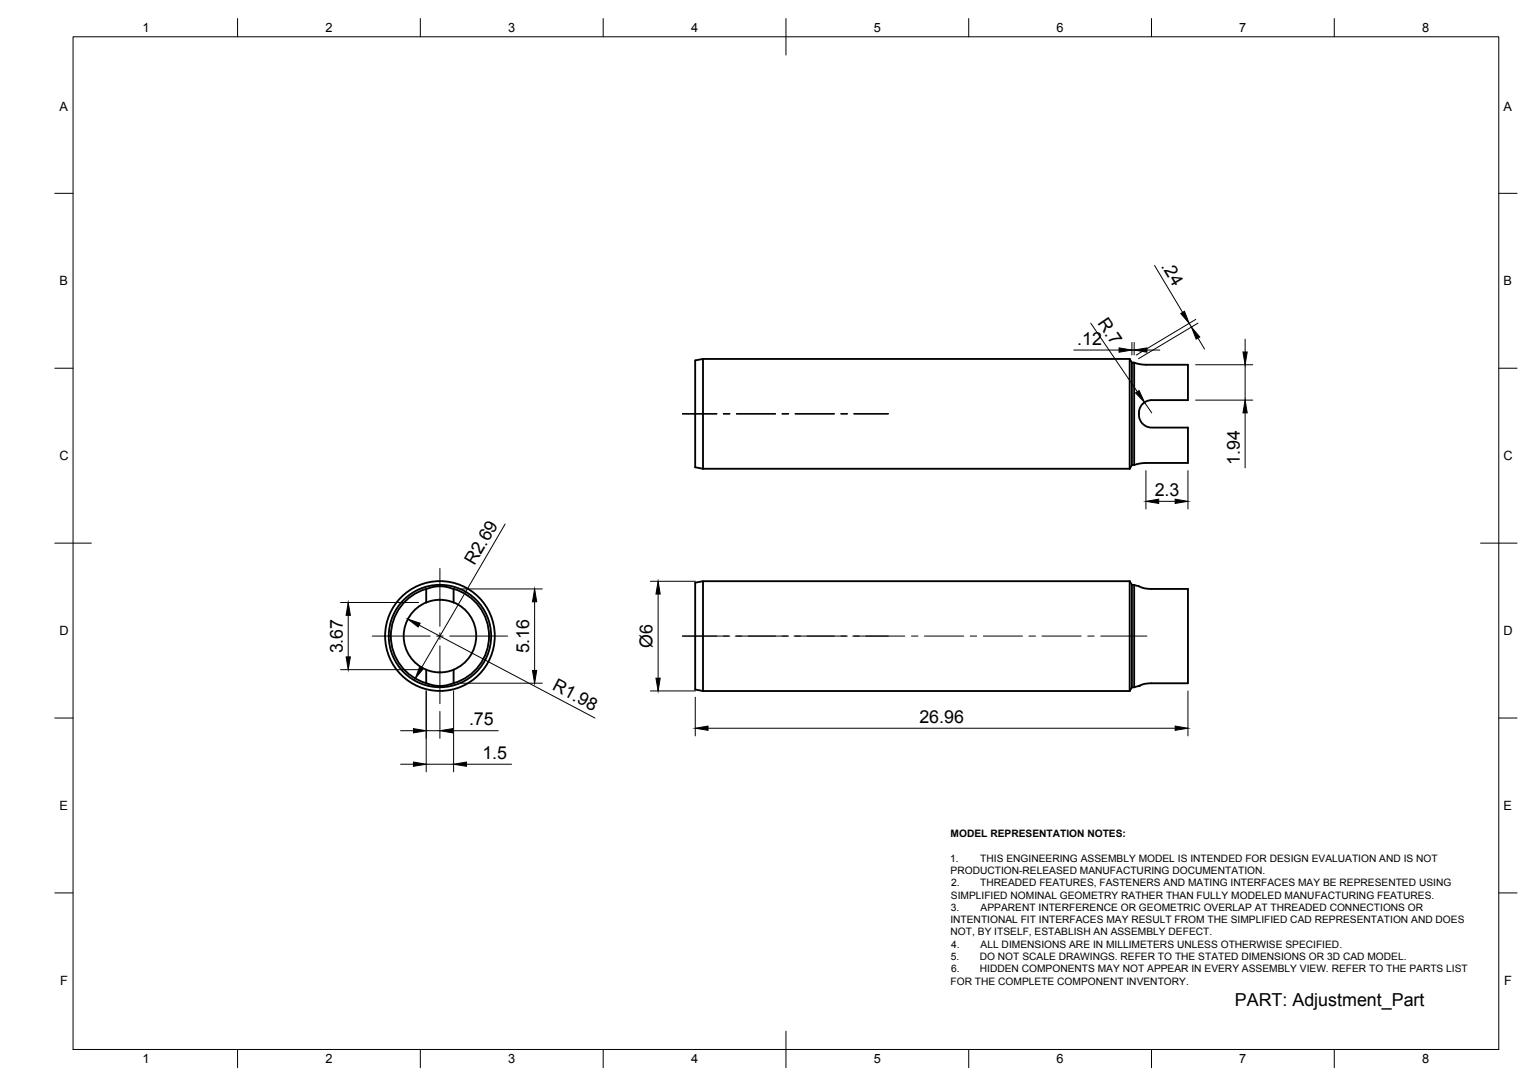
ISO-10303-21;
HEADER;
/* Generated by software containing ST-Developer
 * from STEP Tools, Inc. (www.steptools.com) 
 */

FILE_DESCRIPTION(
/* description */ (''),
/* implementation_level */ '2;1');

FILE_NAME(
/* name */ 'Adjustment_Part.step',
/* time_stamp */ '2026-10-05T00:51:14-07:00',
/* author */ (''),
/* organization */ (''),
/* preprocessor_version */ 'ST-DEVELOPER v20.2',
/* originating_system */ 'Autodesk Translation Framework v15.15.0.0',
/* authorisation */ '');

FILE_SCHEMA (('AUTOMOTIVE_DESIGN { 1 0 10303 214 3 1 1 }'));
ENDSEC;

DATA;
#10=MECHANICAL_DESIGN_GEOMETRIC_PRESENTATION_REPRESENTATION('',(#393),#4613);
#43=TOROIDAL_SURFACE('',#1858,4.57788729236058,1.89228053659161);
#64=CONICAL_SURFACE('',#1877,2.89950556638236,1.03144708645266);
#65=CONICAL_SURFACE('',#1881,2.96124530227324,0.181516066311168);
#89=FACE_BOUND('',#627,.T.);
#90=FACE_BOUND('',#633,.T.);
#120=PLANE('',#1842);
#121=PLANE('',#1843);
#122=PLANE('',#1845);
#123=PLANE('',#1848);
#124=PLANE('',#1850);
#125=PLANE('',#1852);
#126=PLANE('',#1871);
#127=PLANE('',#1872);
#128=PLANE('',#1873);
#129=PLANE('',#1883);
#153=B_SPLINE_CURVE_WITH_KNOTS('',3,(#4375,#4376,#4377,#4378,#4379,#4380),
 .UNSPECIFIED.,.F.,.F.,(4,2,4),(0.,0.0265093466366244,0.0315326488828016),
 .UNSPECIFIED.);
#154=B_SPLINE_CURVE_WITH_KNOTS('',3,(#4382,#4383,#4384,#4385,#4386,#4387,
#4388,#4389,#4390,#4391),.UNSPECIFIED.,.F.,.F.,(4,2,2,2,4),(-0.106715130399001,
-0.0799992414062105,-0.0532833524134197,-0.0266416762067098,0.),
 .UNSPECIFIED.);
#155=B_SPLINE_CURVE_WITH_KNOTS('',3,(#4394,#4395,#4396,#4397,#4398,#4399,
#4400,#4401,#4402,#4403,#4404,#4405,#4406),.UNSPECIFIED.,.F.,.F.,(4,2,2,
2,3,4),(0.378639974335924,0.39855724329992,0.425776827887283,0.447703205216881,
0.457107149533339,0.457130414187804),.UNSPECIFIED.);
#156=B_SPLINE_CURVE_WITH_KNOTS('',3,(#4424,#4425,#4426,#4427,#4428,#4429,
#4430,#4431,#4432,#4433,#4434,#4435,#4436),.UNSPECIFIED.,.F.,.F.,(4,3,2,
2,2,4),(0.457052713610798,0.457075978112808,0.477097828431014,0.502267294711213,
0.530728459336765,0.53557163395288),.UNSPECIFIED.);
#157=B_SPLINE_CURVE_WITH_KNOTS('',3,(#4437,#4438,#4439,#4440,#4441,#4442,
#4443,#4444,#4445,#4446),.UNSPECIFIED.,.F.,.F.,(4,2,2,2,4),(-0.212983885016079,
-0.186342208809369,-0.159700532602659,-0.132984643609868,-0.106268754617077),
 .UNSPECIFIED.);
#158=B_SPLINE_CURVE_WITH_KNOTS('',3,(#4447,#4448,#4449,#4450,#4451,#4452),
 .UNSPECIFIED.,.F.,.F.,(4,2,4),(0.180491212128822,0.185514514374999,0.212023861011624),
 .UNSPECIFIED.);
#159=B_SPLINE_CURVE_WITH_KNOTS('',3,(#4465,#4466,#4467,#4468,#4469,#4470,
#4471,#4472,#4473,#4474),.UNSPECIFIED.,.F.,.F.,(4,2,2,2,4),(0.152701408415346,
0.169165149472481,0.195857989456366,0.218518872787138,0.230918738867668),
 .UNSPECIFIED.);
#160=B_SPLINE_CURVE_WITH_KNOTS('',3,(#4475,#4476,#4477,#4478,#4479,#4480),
 .UNSPECIFIED.,.F.,.F.,(4,2,4),(0.212023861011624,0.238533207648248,0.243556509894426),
 .UNSPECIFIED.);
#161=B_SPLINE_CURVE_WITH_KNOTS('',3,(#4482,#4483,#4484,#4485,#4486,#4487,
#4488,#4489,#4490,#4491),.UNSPECIFIED.,.F.,.F.,(4,2,2,2,4),(-0.319699015415081,
-0.29298312642229,-0.266267237429499,-0.239625561222789,-0.212983885016079),
 .UNSPECIFIED.);
#162=B_SPLINE_CURVE_WITH_KNOTS('',3,(#4505,#4506,#4507,#4508,#4509,#4510),
 .UNSPECIFIED.,.F.,.F.,(4,2,4),(0.392515073140443,0.39753837538662,0.424047722023245),
 .UNSPECIFIED.);
#163=B_SPLINE_CURVE_WITH_KNOTS('',3,(#4511,#4512,#4513,#4514,#4515,#4516,
#4517,#4518,#4519,#4520),.UNSPECIFIED.,.F.,.F.,(4,2,2,2,4),(0.224352648954622,
0.240815002701601,0.264724046908964,0.293460711591788,0.30255788453281),
 .UNSPECIFIED.);
#164=B_SPLINE_CURVE_WITH_KNOTS('',3,(#4521,#4522,#4523,#4524,#4525,#4526,
#4527,#4528,#4529,#4530),.UNSPECIFIED.,.F.,.F.,(4,2,2,2,4),(-0.425967770032155,
-0.399326093825445,-0.372684417618735,-0.345968528625944,-0.319252639633153),
 .UNSPECIFIED.);
#220=LINE('',#4358,#303);
#221=LINE('',#4360,#304);
#222=LINE('',#4362,#305);
#223=LINE('',#4363,#306);
#224=LINE('',#4367,#307);
#225=LINE('',#4369,#308);
#226=LINE('',#4371,#309);
#227=LINE('',#4372,#310);
#228=LINE('',#4393,#311);
#229=LINE('',#4412,#312);
#230=LINE('',#4416,#313);
#231=LINE('',#4418,#314);
#232=LINE('',#4420,#315);
#233=LINE('',#4421,#316);
#234=LINE('',#4456,#317);
#235=LINE('',#4458,#318);
#236=LINE('',#4460,#319);
#237=LINE('',#4461,#320);
#238=LINE('',#4492,#321);
#239=LINE('',#4501,#322);
#240=LINE('',#4539,#323);
#241=LINE('',#4555,#324);
#242=LINE('',#4559,#325);
#243=LINE('',#4563,#326);
#244=LINE('',#4566,#327);
#245=LINE('',#4572,#328);
#303=VECTOR('',#2261,10.);
#304=VECTOR('',#2262,10.);
#305=VECTOR('',#2263,10.);
#306=VECTOR('',#2264,10.);
#307=VECTOR('',#2267,10.);
#308=VECTOR('',#2268,10.);
#309=VECTOR('',#2269,10.);
#310=VECTOR('',#2270,10.);
#311=VECTOR('',#2273,10.);
#312=VECTOR('',#2280,10.);
#313=VECTOR('',#2283,10.);
#314=VECTOR('',#2284,10.);
#315=VECTOR('',#2285,10.);
#316=VECTOR('',#2286,10.);
#317=VECTOR('',#2291,10.);
#318=VECTOR('',#2292,10.);
#319=VECTOR('',#2293,10.);
#320=VECTOR('',#2294,10.);
#321=VECTOR('',#2297,10.);
#322=VECTOR('',#2306,10.);
#323=VECTOR('',#2323,1.9840612380693);
#324=VECTOR('',#2350,2.79839874569029);
#325=VECTOR('',#2355,2.89950556638236);
#326=VECTOR('',#2360,3.00061238707443);
#327=VECTOR('',#2363,2.96124530227324);
#328=VECTOR('',#2372,2.3164003912567);
#360=CYLINDRICAL_SURFACE('',#1844,0.699999999999994);
#361=CYLINDRICAL_SURFACE('',#1849,0.699999999999998);
#362=CYLINDRICAL_SURFACE('',#1851,0.699999999999998);
#363=CYLINDRICAL_SURFACE('',#1857,0.699999999999994);
#364=CYLINDRICAL_SURFACE('',#1863,1.9840612380693);
#365=CYLINDRICAL_SURFACE('',#1867,2.68560675576897);
#366=CYLINDRICAL_SURFACE('',#1869,2.68560675576897);
#367=CYLINDRICAL_SURFACE('',#1875,2.79839874569029);
#368=CYLINDRICAL_SURFACE('',#1879,3.00061238707443);
#369=CYLINDRICAL_SURFACE('',#1885,2.3164003912567);
#377=SHAPE_REPRESENTATION_RELATIONSHIP('SRR','None',#4651,#385);
#385=ADVANCED_BREP_SHAPE_REPRESENTATION('',(#401),#4611);
#393=STYLED_ITEM('',(#4695),#401);
#401=MANIFOLD_SOLID_BREP('Body1',#1600);
#482=FACE_OUTER_BOUND('',#610,.T.);
#483=FACE_OUTER_BOUND('',#611,.T.);
#484=FACE_OUTER_BOUND('',#612,.T.);
#485=FACE_OUTER_BOUND('',#613,.T.);
#486=FACE_OUTER_BOUND('',#614,.T.);
#487=FACE_OUTER_BOUND('',#615,.T.);
#488=FACE_OUTER_BOUND('',#616,.T.);
#489=FACE_OUTER_BOUND('',#617,.T.);
#490=FACE_OUTER_BOUND('',#618,.T.);
#491=FACE_OUTER_BOUND('',#619,.T.);
#492=FACE_OUTER_BOUND('',#620,.T.);
#493=FACE_OUTER_BOUND('',#621,.T.);
#494=FACE_OUTER_BOUND('',#622,.T.);
#495=FACE_OUTER_BOUND('',#623,.T.);
#496=FACE_OUTER_BOUND('',#624,.T.);
#497=FACE_OUTER_BOUND('',#625,.T.);
#498=FACE_OUTER_BOUND('',#626,.T.);
#499=FACE_OUTER_BOUND('',#628,.T.);
#500=FACE_OUTER_BOUND('',#629,.T.);
#501=FACE_OUTER_BOUND('',#630,.T.);
#502=FACE_OUTER_BOUND('',#631,.T.);
#503=FACE_OUTER_BOUND('',#632,.T.);
#504=FACE_OUTER_BOUND('',#634,.T.);
#610=EDGE_LOOP('',(#1359,#1360,#1361,#1362));
#611=EDGE_LOOP('',(#1363,#1364,#1365,#1366));
#612=EDGE_LOOP('',(#1367,#1368,#1369,#1370,#1371));
#613=EDGE_LOOP('',(#1372,#1373,#1374,#1375));
#614=EDGE_LOOP('',(#1376,#1377,#1378,#1379));
#615=EDGE_LOOP('',(#1380,#1381,#1382,#1383,#1384));
#616=EDGE_LOOP('',(#1385,#1386,#1387,#1388));
#617=EDGE_LOOP('',(#1389,#1390,#1391,#1392,#1393));
#618=EDGE_LOOP('',(#1394,#1395,#1396,#1397,#1398,#1399));
#619=EDGE_LOOP('',(#1400,#1401,#1402,#1403,#1404));
#620=EDGE_LOOP('',(#1405,#1406,#1407,#1408,#1409,#1410,#1411,#1412,#1413,
#1414,#1415,#1416));
#621=EDGE_LOOP('',(#1417,#1418,#1419,#1420,#1421,#1422,#1423,#1424,#1425,
#1426,#1427,#1428,#1429,#1430,#1431,#1432));
#622=EDGE_LOOP('',(#1433,#1434,#1435,#1436,#1437,#1438));
#623=EDGE_LOOP('',(#1439,#1440,#1441,#1442,#1443,#1444));
#624=EDGE_LOOP('',(#1445,#1446,#1447,#1448));
#625=EDGE_LOOP('',(#1449,#1450,#1451,#1452));
#626=EDGE_LOOP('',(#1453));
#627=EDGE_LOOP('',(#1454));
#628=EDGE_LOOP('',(#1455,#1456,#1457,#1458));
#629=EDGE_LOOP('',(#1459,#1460,#1461,#1462));
#630=EDGE_LOOP('',(#1463,#1464,#1465,#1466));
#631=EDGE_LOOP('',(#1467,#1468,#1469,#1470));
#632=EDGE_LOOP('',(#1471));
#633=EDGE_LOOP('',(#1472));
#634=EDGE_LOOP('',(#1473,#1474,#1475,#1476));
#707=CIRCLE('',#1846,2.7248783394621);
#708=CIRCLE('',#1847,1.9840612380693);
#709=CIRCLE('',#1853,2.7248783394621);
#710=CIRCLE('',#1854,1.9840612380693);
#711=CIRCLE('',#1855,1.9840612380693);
#712=CIRCLE('',#1856,2.7248783394621);
#713=CIRCLE('',#1859,2.79839874569029);
#714=CIRCLE('',#1860,1.89228053659161);
#715=CIRCLE('',#1861,2.68560675576897);
#716=CIRCLE('',#1862,2.68560675576897);
#717=CIRCLE('',#1864,1.9840612380693);
#718=CIRCLE('',#1865,1.9840612380693);
#719=CIRCLE('',#1866,1.9840612380693);
#720=CIRCLE('',#1868,2.68560675576897);
#721=CIRCLE('',#1870,2.68560675576897);
#722=CIRCLE('',#1874,2.3164003912567);
#723=CIRCLE('',#1876,2.79839874569029);
#724=CIRCLE('',#1878,3.00061238707443);
#725=CIRCLE('',#1880,3.00061238707443);
#726=CIRCLE('',#1882,2.92187821747206);
#727=CIRCLE('',#1884,2.3164003912567);
#822=VERTEX_POINT('',#4356);
#823=VERTEX_POINT('',#4357);
#824=VERTEX_POINT('',#4359);
#825=VERTEX_POINT('',#4361);
#826=VERTEX_POINT('',#4365);
#827=VERTEX_POINT('',#4366);
#828=VERTEX_POINT('',#4368);
#829=VERTEX_POINT('',#4370);
#830=VERTEX_POINT('',#4374);
#831=VERTEX_POINT('',#4381);
#832=VERTEX_POINT('',#4392);
#833=VERTEX_POINT('',#4408);
#834=VERTEX_POINT('',#4410);
#835=VERTEX_POINT('',#4414);
#836=VERTEX_POINT('',#4415);
#837=VERTEX_POINT('',#4417);
#838=VERTEX_POINT('',#4419);
#839=VERTEX_POINT('',#4423);
#840=VERTEX_POINT('',#4454);
#841=VERTEX_POINT('',#4455);
#842=VERTEX_POINT('',#4457);
#843=VERTEX_POINT('',#4459);
#844=VERTEX_POINT('',#4463);
#845=VERTEX_POINT('',#4464);
#846=VERTEX_POINT('',#4481);
#847=VERTEX_POINT('',#4494);
#848=VERTEX_POINT('',#4496);
#849=VERTEX_POINT('',#4498);
#850=VERTEX_POINT('',#4500);
#851=VERTEX_POINT('',#4504);
#852=VERTEX_POINT('',#4532);
#853=VERTEX_POINT('',#4538);
#854=VERTEX_POINT('',#4550);
#855=VERTEX_POINT('',#4553);
#856=VERTEX_POINT('',#4557);
#857=VERTEX_POINT('',#4561);
#858=VERTEX_POINT('',#4565);
#859=VERTEX_POINT('',#4569);
#1007=EDGE_CURVE('',#822,#823,#220,.T.);
#1008=EDGE_CURVE('',#824,#822,#221,.T.);
#1009=EDGE_CURVE('',#825,#824,#222,.T.);
#1010=EDGE_CURVE('',#825,#823,#223,.T.);
#1011=EDGE_CURVE('',#826,#827,#224,.T.);
#1012=EDGE_CURVE('',#826,#828,#225,.T.);
#1013=EDGE_CURVE('',#829,#828,#226,.T.);
#1014=EDGE_CURVE('',#827,#829,#227,.T.);
#1015=EDGE_CURVE('',#823,#830,#153,.T.);
#1016=EDGE_CURVE('',#831,#825,#154,.T.);
#1017=EDGE_CURVE('',#832,#831,#228,.T.);
#1018=EDGE_CURVE('',#830,#832,#155,.T.);
#1019=EDGE_CURVE('',#832,#833,#707,.T.);
#1020=EDGE_CURVE('',#834,#831,#708,.T.);
#1021=EDGE_CURVE('',#833,#834,#229,.T.);
#1022=EDGE_CURVE('',#835,#836,#230,.T.);
#1023=EDGE_CURVE('',#835,#837,#231,.T.);
#1024=EDGE_CURVE('',#838,#837,#232,.T.);
#1025=EDGE_CURVE('',#836,#838,#233,.T.);
#1026=EDGE_CURVE('',#833,#839,#156,.T.);
#1027=EDGE_CURVE('',#837,#834,#157,.T.);
#1028=EDGE_CURVE('',#839,#835,#158,.T.);
#1029=EDGE_CURVE('',#840,#841,#234,.T.);
#1030=EDGE_CURVE('',#842,#840,#235,.T.);
#1031=EDGE_CURVE('',#843,#842,#236,.T.);
#1032=EDGE_CURVE('',#843,#841,#237,.T.);
#1033=EDGE_CURVE('',#844,#845,#159,.T.);
#1034=EDGE_CURVE('',#841,#844,#160,.T.);
#1035=EDGE_CURVE('',#846,#843,#161,.T.);
#1036=EDGE_CURVE('',#846,#845,#238,.T.);
#1037=EDGE_CURVE('',#845,#847,#709,.T.);
#1038=EDGE_CURVE('',#848,#846,#710,.T.);
#1039=EDGE_CURVE('',#849,#848,#711,.T.);
#1040=EDGE_CURVE('',#849,#850,#239,.T.);
#1041=EDGE_CURVE('',#847,#850,#712,.T.);
#1042=EDGE_CURVE('',#851,#826,#162,.T.);
#1043=EDGE_CURVE('',#850,#851,#163,.T.);
#1044=EDGE_CURVE('',#828,#849,#164,.T.);
#1045=EDGE_CURVE('',#852,#852,#713,.T.);
#1046=EDGE_CURVE('',#852,#847,#714,.T.);
#1047=EDGE_CURVE('',#851,#830,#715,.T.);
#1048=EDGE_CURVE('',#839,#844,#716,.T.);
#1049=EDGE_CURVE('',#848,#853,#240,.T.);
#1050=EDGE_CURVE('',#853,#853,#717,.T.);
#1051=EDGE_CURVE('',#838,#842,#718,.T.);
#1052=EDGE_CURVE('',#829,#824,#719,.T.);
#1053=EDGE_CURVE('',#836,#840,#720,.T.);
#1054=EDGE_CURVE('',#827,#822,#721,.T.);
#1055=EDGE_CURVE('',#854,#854,#722,.T.);
#1056=EDGE_CURVE('',#855,#855,#723,.T.);
#1057=EDGE_CURVE('',#855,#852,#241,.T.);
#1058=EDGE_CURVE('',#856,#856,#724,.T.);
#1059=EDGE_CURVE('',#856,#855,#242,.T.);
#1060=EDGE_CURVE('',#857,#857,#725,.T.);
#1061=EDGE_CURVE('',#857,#856,#243,.T.);
#1062=EDGE_CURVE('',#857,#858,#244,.T.);
#1063=EDGE_CURVE('',#858,#858,#726,.T.);
#1064=EDGE_CURVE('',#859,#859,#727,.T.);
#1065=EDGE_CURVE('',#854,#859,#245,.T.);
#1359=ORIENTED_EDGE('',*,*,#1007,.F.);
#1360=ORIENTED_EDGE('',*,*,#1008,.F.);
#1361=ORIENTED_EDGE('',*,*,#1009,.F.);
#1362=ORIENTED_EDGE('',*,*,#1010,.T.);
#1363=ORIENTED_EDGE('',*,*,#1011,.F.);
#1364=ORIENTED_EDGE('',*,*,#1012,.T.);
#1365=ORIENTED_EDGE('',*,*,#1013,.F.);
#1366=ORIENTED_EDGE('',*,*,#1014,.F.);
#1367=ORIENTED_EDGE('',*,*,#1015,.F.);
#1368=ORIENTED_EDGE('',*,*,#1010,.F.);
#1369=ORIENTED_EDGE('',*,*,#1016,.F.);
#1370=ORIENTED_EDGE('',*,*,#1017,.F.);
#1371=ORIENTED_EDGE('',*,*,#1018,.F.);
#1372=ORIENTED_EDGE('',*,*,#1019,.F.);
#1373=ORIENTED_EDGE('',*,*,#1017,.T.);
#1374=ORIENTED_EDGE('',*,*,#1020,.F.);
#1375=ORIENTED_EDGE('',*,*,#1021,.F.);
#1376=ORIENTED_EDGE('',*,*,#1022,.F.);
#1377=ORIENTED_EDGE('',*,*,#1023,.T.);
#1378=ORIENTED_EDGE('',*,*,#1024,.F.);
#1379=ORIENTED_EDGE('',*,*,#1025,.F.);
#1380=ORIENTED_EDGE('',*,*,#1026,.F.);
#1381=ORIENTED_EDGE('',*,*,#1021,.T.);
#1382=ORIENTED_EDGE('',*,*,#1027,.F.);
#1383=ORIENTED_EDGE('',*,*,#1023,.F.);
#1384=ORIENTED_EDGE('',*,*,#1028,.F.);
#1385=ORIENTED_EDGE('',*,*,#1029,.F.);
#1386=ORIENTED_EDGE('',*,*,#1030,.F.);
#1387=ORIENTED_EDGE('',*,*,#1031,.F.);
#1388=ORIENTED_EDGE('',*,*,#1032,.T.);
#1389=ORIENTED_EDGE('',*,*,#1033,.F.);
#1390=ORIENTED_EDGE('',*,*,#1034,.F.);
#1391=ORIENTED_EDGE('',*,*,#1032,.F.);
#1392=ORIENTED_EDGE('',*,*,#1035,.F.);
#1393=ORIENTED_EDGE('',*,*,#1036,.T.);
#1394=ORIENTED_EDGE('',*,*,#1037,.F.);
#1395=ORIENTED_EDGE('',*,*,#1036,.F.);
#1396=ORIENTED_EDGE('',*,*,#1038,.F.);
#1397=ORIENTED_EDGE('',*,*,#1039,.F.);
#1398=ORIENTED_EDGE('',*,*,#1040,.T.);
#1399=ORIENTED_EDGE('',*,*,#1041,.F.);
#1400=ORIENTED_EDGE('',*,*,#1042,.F.);
#1401=ORIENTED_EDGE('',*,*,#1043,.F.);
#1402=ORIENTED_EDGE('',*,*,#1040,.F.);
#1403=ORIENTED_EDGE('',*,*,#1044,.F.);
#1404=ORIENTED_EDGE('',*,*,#1012,.F.);
#1405=ORIENTED_EDGE('',*,*,#1045,.F.);
#1406=ORIENTED_EDGE('',*,*,#1046,.T.);
#1407=ORIENTED_EDGE('',*,*,#1041,.T.);
#1408=ORIENTED_EDGE('',*,*,#1043,.T.);
#1409=ORIENTED_EDGE('',*,*,#1047,.T.);
#1410=ORIENTED_EDGE('',*,*,#1018,.T.);
#1411=ORIENTED_EDGE('',*,*,#1019,.T.);
#1412=ORIENTED_EDGE('',*,*,#1026,.T.);
#1413=ORIENTED_EDGE('',*,*,#1048,.T.);
#1414=ORIENTED_EDGE('',*,*,#1033,.T.);
#1415=ORIENTED_EDGE('',*,*,#1037,.T.);
#1416=ORIENTED_EDGE('',*,*,#1046,.F.);
#1417=ORIENTED_EDGE('',*,*,#1039,.T.);
#1418=ORIENTED_EDGE('',*,*,#1049,.T.);
#1419=ORIENTED_EDGE('',*,*,#1050,.T.);
#1420=ORIENTED_EDGE('',*,*,#1049,.F.);
#1421=ORIENTED_EDGE('',*,*,#1038,.T.);
#1422=ORIENTED_EDGE('',*,*,#1035,.T.);
#1423=ORIENTED_EDGE('',*,*,#1031,.T.);
#1424=ORIENTED_EDGE('',*,*,#1051,.F.);
#1425=ORIENTED_EDGE('',*,*,#1024,.T.);
#1426=ORIENTED_EDGE('',*,*,#1027,.T.);
#1427=ORIENTED_EDGE('',*,*,#1020,.T.);
#1428=ORIENTED_EDGE('',*,*,#1016,.T.);
#1429=ORIENTED_EDGE('',*,*,#1009,.T.);
#1430=ORIENTED_EDGE('',*,*,#1052,.F.);
#1431=ORIENTED_EDGE('',*,*,#1013,.T.);
#1432=ORIENTED_EDGE('',*,*,#1044,.T.);
#1433=ORIENTED_EDGE('',*,*,#1034,.T.);
#1434=ORIENTED_EDGE('',*,*,#1048,.F.);
#1435=ORIENTED_EDGE('',*,*,#1028,.T.);
#1436=ORIENTED_EDGE('',*,*,#1022,.T.);
#1437=ORIENTED_EDGE('',*,*,#1053,.T.);
#1438=ORIENTED_EDGE('',*,*,#1029,.T.);
#1439=ORIENTED_EDGE('',*,*,#1042,.T.);
#1440=ORIENTED_EDGE('',*,*,#1011,.T.);
#1441=ORIENTED_EDGE('',*,*,#1054,.T.);
#1442=ORIENTED_EDGE('',*,*,#1007,.T.);
#1443=ORIENTED_EDGE('',*,*,#1015,.T.);
#1444=ORIENTED_EDGE('',*,*,#1047,.F.);
#1445=ORIENTED_EDGE('',*,*,#1030,.T.);
#1446=ORIENTED_EDGE('',*,*,#1053,.F.);
#1447=ORIENTED_EDGE('',*,*,#1025,.T.);
#1448=ORIENTED_EDGE('',*,*,#1051,.T.);
#1449=ORIENTED_EDGE('',*,*,#1014,.T.);
#1450=ORIENTED_EDGE('',*,*,#1052,.T.);
#1451=ORIENTED_EDGE('',*,*,#1008,.T.);
#1452=ORIENTED_EDGE('',*,*,#1054,.F.);
#1453=ORIENTED_EDGE('',*,*,#1055,.T.);
#1454=ORIENTED_EDGE('',*,*,#1050,.F.);
#1455=ORIENTED_EDGE('',*,*,#1056,.F.);
#1456=ORIENTED_EDGE('',*,*,#1057,.T.);
#1457=ORIENTED_EDGE('',*,*,#1045,.T.);
#1458=ORIENTED_EDGE('',*,*,#1057,.F.);
#1459=ORIENTED_EDGE('',*,*,#1058,.F.);
#1460=ORIENTED_EDGE('',*,*,#1059,.T.);
#1461=ORIENTED_EDGE('',*,*,#1056,.T.);
#1462=ORIENTED_EDGE('',*,*,#1059,.F.);
#1463=ORIENTED_EDGE('',*,*,#1060,.F.);
#1464=ORIENTED_EDGE('',*,*,#1061,.T.);
#1465=ORIENTED_EDGE('',*,*,#1058,.T.);
#1466=ORIENTED_EDGE('',*,*,#1061,.F.);
#1467=ORIENTED_EDGE('',*,*,#1060,.T.);
#1468=ORIENTED_EDGE('',*,*,#1062,.T.);
#1469=ORIENTED_EDGE('',*,*,#1063,.F.);
#1470=ORIENTED_EDGE('',*,*,#1062,.F.);
#1471=ORIENTED_EDGE('',*,*,#1063,.T.);
#1472=ORIENTED_EDGE('',*,*,#1064,.F.);
#1473=ORIENTED_EDGE('',*,*,#1055,.F.);
#1474=ORIENTED_EDGE('',*,*,#1065,.T.);
#1475=ORIENTED_EDGE('',*,*,#1064,.T.);
#1476=ORIENTED_EDGE('',*,*,#1065,.F.);
#1567=ADVANCED_FACE('',(#482),#120,.F.);
#1568=ADVANCED_FACE('',(#483),#121,.F.);
#1569=ADVANCED_FACE('',(#484),#360,.F.);
#1570=ADVANCED_FACE('',(#485),#122,.F.);
#1571=ADVANCED_FACE('',(#486),#123,.F.);
#1572=ADVANCED_FACE('',(#487),#361,.F.);
#1573=ADVANCED_FACE('',(#488),#124,.F.);
#1574=ADVANCED_FACE('',(#489),#362,.F.);
#1575=ADVANCED_FACE('',(#490),#125,.F.);
#1576=ADVANCED_FACE('',(#491),#363,.F.);
#1577=ADVANCED_FACE('',(#492),#43,.F.);
#1578=ADVANCED_FACE('',(#493),#364,.F.);
#1579=ADVANCED_FACE('',(#494),#365,.T.);
#1580=ADVANCED_FACE('',(#495),#366,.T.);
#1581=ADVANCED_FACE('',(#496),#126,.T.);
#1582=ADVANCED_FACE('',(#497),#127,.T.);
#1583=ADVANCED_FACE('',(#498,#89),#128,.T.);
#1584=ADVANCED_FACE('',(#499),#367,.T.);
#1585=ADVANCED_FACE('',(#500),#64,.T.);
#1586=ADVANCED_FACE('',(#501),#368,.T.);
#1587=ADVANCED_FACE('',(#502),#65,.T.);
#1588=ADVANCED_FACE('',(#503,#90),#129,.T.);
#1589=ADVANCED_FACE('',(#504),#369,.F.);
#1600=CLOSED_SHELL('',(#1567,#1568,#1569,#1570,#1571,#1572,#1573,#1574,
#1575,#1576,#1577,#1578,#1579,#1580,#1581,#1582,#1583,#1584,#1585,#1586,
#1587,#1588,#1589));
#1841=AXIS2_PLACEMENT_3D('',#4354,#2257,#2258);
#1842=AXIS2_PLACEMENT_3D('',#4355,#2259,#2260);
#1843=AXIS2_PLACEMENT_3D('',#4364,#2265,#2266);
#1844=AXIS2_PLACEMENT_3D('',#4373,#2271,#2272);
#1845=AXIS2_PLACEMENT_3D('',#4407,#2274,#2275);
#1846=AXIS2_PLACEMENT_3D('',#4409,#2276,#2277);
#1847=AXIS2_PLACEMENT_3D('',#4411,#2278,#2279);
#1848=AXIS2_PLACEMENT_3D('',#4413,#2281,#2282);
#1849=AXIS2_PLACEMENT_3D('',#4422,#2287,#2288);
#1850=AXIS2_PLACEMENT_3D('',#4453,#2289,#2290);
#1851=AXIS2_PLACEMENT_3D('',#4462,#2295,#2296);
#1852=AXIS2_PLACEMENT_3D('',#4493,#2298,#2299);
#1853=AXIS2_PLACEMENT_3D('',#4495,#2300,#2301);
#1854=AXIS2_PLACEMENT_3D('',#4497,#2302,#2303);
#1855=AXIS2_PLACEMENT_3D('',#4499,#2304,#2305);
#1856=AXIS2_PLACEMENT_3D('',#4502,#2307,#2308);
#1857=AXIS2_PLACEMENT_3D('',#4503,#2309,#2310);
#1858=AXIS2_PLACEMENT_3D('',#4531,#2311,#2312);
#1859=AXIS2_PLACEMENT_3D('',#4533,#2313,#2314);
#1860=AXIS2_PLACEMENT_3D('',#4534,#2315,#2316);
#1861=AXIS2_PLACEMENT_3D('',#4535,#2317,#2318);
#1862=AXIS2_PLACEMENT_3D('',#4536,#2319,#2320);
#1863=AXIS2_PLACEMENT_3D('',#4537,#2321,#2322);
#1864=AXIS2_PLACEMENT_3D('',#4540,#2324,#2325);
#1865=AXIS2_PLACEMENT_3D('',#4541,#2326,#2327);
#1866=AXIS2_PLACEMENT_3D('',#4542,#2328,#2329);
#1867=AXIS2_PLACEMENT_3D('',#4543,#2330,#2331);
#1868=AXIS2_PLACEMENT_3D('',#4544,#2332,#2333);
#1869=AXIS2_PLACEMENT_3D('',#4545,#2334,#2335);
#1870=AXIS2_PLACEMENT_3D('',#4546,#2336,#2337);
#1871=AXIS2_PLACEMENT_3D('',#4547,#2338,#2339);
#1872=AXIS2_PLACEMENT_3D('',#4548,#2340,#2341);
#1873=AXIS2_PLACEMENT_3D('',#4549,#2342,#2343);
#1874=AXIS2_PLACEMENT_3D('',#4551,#2344,#2345);
#1875=AXIS2_PLACEMENT_3D('',#4552,#2346,#2347);
#1876=AXIS2_PLACEMENT_3D('',#4554,#2348,#2349);
#1877=AXIS2_PLACEMENT_3D('',#4556,#2351,#2352);
#1878=AXIS2_PLACEMENT_3D('',#4558,#2353,#2354);
#1879=AXIS2_PLACEMENT_3D('',#4560,#2356,#2357);
#1880=AXIS2_PLACEMENT_3D('',#4562,#2358,#2359);
#1881=AXIS2_PLACEMENT_3D('',#4564,#2361,#2362);
#1882=AXIS2_PLACEMENT_3D('',#4567,#2364,#2365);
#1883=AXIS2_PLACEMENT_3D('',#4568,#2366,#2367);
#1884=AXIS2_PLACEMENT_3D('',#4570,#2368,#2369);
#1885=AXIS2_PLACEMENT_3D('',#4571,#2370,#2371);
#2257=DIRECTION('axis',(0.,0.,1.));
#2258=DIRECTION('refdir',(1.,0.,0.));
#2259=DIRECTION('center_axis',(1.57016756309984E-16,-1.,0.));
#2260=DIRECTION('ref_axis',(1.,1.57016756309984E-16,0.));
#2261=DIRECTION('',(1.,0.,0.));
#2262=DIRECTION('',(0.,0.,-1.));
#2263=DIRECTION('',(-1.,0.,0.));
#2264=DIRECTION('',(0.,0.,-1.));
#2265=DIRECTION('center_axis',(1.57016756309984E-16,-1.,0.));
#2266=DIRECTION('ref_axis',(1.,1.57016756309984E-16,0.));
#2267=DIRECTION('',(-1.,0.,0.));
#2268=DIRECTION('',(0.,0.,-1.));
#2269=DIRECTION('',(1.,0.,0.));
#2270=DIRECTION('',(0.,0.,-1.));
#2271=DIRECTION('center_axis',(0.,0.,1.));
#2272=DIRECTION('ref_axis',(-6.34413156928666E-15,-1.,0.));
#2273=DIRECTION('',(0.,0.,1.));
#2274=DIRECTION('center_axis',(1.,0.,0.));
#2275=DIRECTION('ref_axis',(0.,1.,0.));
#2276=DIRECTION('center_axis',(1.,0.,0.));
#2277=DIRECTION('ref_axis',(0.,0.,-1.));
#2278=DIRECTION('center_axis',(-1.,0.,0.));
#2279=DIRECTION('ref_axis',(0.,0.,-1.));
#2280=DIRECTION('',(0.,0.,1.));
#2281=DIRECTION('center_axis',(-2.35525134464976E-16,1.,0.));
#2282=DIRECTION('ref_axis',(-1.,-2.35525134464976E-16,0.));
#2283=DIRECTION('',(-1.,0.,0.));
#2284=DIRECTION('',(0.,0.,1.));
#2285=DIRECTION('',(1.,0.,0.));
#2286=DIRECTION('',(0.,0.,1.));
#2287=DIRECTION('center_axis',(0.,0.,1.));
#2288=DIRECTION('ref_axis',(1.,1.11517937741366E-16,0.));
#2289=DIRECTION('center_axis',(-2.35525134464976E-16,1.,0.));
#2290=DIRECTION('ref_axis',(-1.,-2.35525134464976E-16,0.));
#2291=DIRECTION('',(1.,0.,0.));
#2292=DIRECTION('',(0.,0.,1.));
#2293=DIRECTION('',(-1.,0.,0.));
#2294=DIRECTION('',(0.,0.,1.));
#2295=DIRECTION('center_axis',(0.,0.,1.));
#2296=DIRECTION('ref_axis',(1.,1.11517937741366E-16,0.));
#2297=DIRECTION('',(0.,0.,1.));
#2298=DIRECTION('center_axis',(1.,0.,0.));
#2299=DIRECTION('ref_axis',(0.,1.,0.));
#2300=DIRECTION('center_axis',(1.,0.,0.));
#2301=DIRECTION('ref_axis',(0.,0.,-1.));
#2302=DIRECTION('center_axis',(-1.,0.,0.));
#2303=DIRECTION('ref_axis',(0.,0.,-1.));
#2304=DIRECTION('center_axis',(-1.,0.,0.));
#2305=DIRECTION('ref_axis',(0.,0.,-1.));
#2306=DIRECTION('',(0.,0.,1.));
#2307=DIRECTION('center_axis',(1.,0.,0.));
#2308=DIRECTION('ref_axis',(0.,0.,-1.));
#2309=DIRECTION('center_axis',(0.,0.,1.));
#2310=DIRECTION('ref_axis',(-6.34413156928666E-15,-1.,0.));
#2311=DIRECTION('center_axis',(1.,0.,0.));
#2312=DIRECTION('ref_axis',(0.,0.,-1.));
#2313=DIRECTION('center_axis',(1.,0.,0.));
#2314=DIRECTION('ref_axis',(0.,0.,-1.));
#2315=DIRECTION('center_axis',(0.,1.,1.22464679914735E-16));
#2316=DIRECTION('ref_axis',(0.,-1.22464679914735E-16,1.));
#2317=DIRECTION('center_axis',(1.,0.,0.));
#2318=DIRECTION('ref_axis',(0.,0.,-1.));
#2319=DIRECTION('center_axis',(1.,0.,0.));
#2320=DIRECTION('ref_axis',(0.,0.,-1.));
#2321=DIRECTION('center_axis',(1.,0.,0.));
#2322=DIRECTION('ref_axis',(0.,0.,-1.));
#2323=DIRECTION('',(1.,0.,0.));
#2324=DIRECTION('center_axis',(1.,0.,0.));
#2325=DIRECTION('ref_axis',(0.,0.,-1.));
#2326=DIRECTION('center_axis',(1.,0.,0.));
#2327=DIRECTION('ref_axis',(0.,0.,-1.));
#2328=DIRECTION('center_axis',(1.,0.,0.));
#2329=DIRECTION('ref_axis',(0.,0.,-1.));
#2330=DIRECTION('center_axis',(1.,0.,0.));
#2331=DIRECTION('ref_axis',(0.,0.,-1.));
#2332=DIRECTION('center_axis',(1.,0.,0.));
#2333=DIRECTION('ref_axis',(0.,0.,-1.));
#2334=DIRECTION('center_axis',(1.,0.,0.));
#2335=DIRECTION('ref_axis',(0.,0.,-1.));
#2336=DIRECTION('center_axis',(1.,0.,0.));
#2337=DIRECTION('ref_axis',(0.,0.,-1.));
#2338=DIRECTION('center_axis',(-1.,0.,0.));
#2339=DIRECTION('ref_axis',(0.,0.,1.));
#2340=DIRECTION('center_axis',(-1.,0.,0.));
#2341=DIRECTION('ref_axis',(0.,0.,1.));
#2342=DIRECTION('center_axis',(1.,0.,0.));
#2343=DIRECTION('ref_axis',(0.,0.,-1.));
#2344=DIRECTION('center_axis',(1.,0.,0.));
#2345=DIRECTION('ref_axis',(0.,0.,-1.));
#2346=DIRECTION('center_axis',(1.,0.,0.));
#2347=DIRECTION('ref_axis',(0.,0.,-1.));
#2348=DIRECTION('center_axis',(1.,0.,0.));
#2349=DIRECTION('ref_axis',(0.,0.,-1.));
#2350=DIRECTION('',(-1.,0.,0.));
#2351=DIRECTION('center_axis',(1.,0.,0.));
#2352=DIRECTION('ref_axis',(0.,0.,-1.));
#2353=DIRECTION('center_axis',(1.,0.,0.));
#2354=DIRECTION('ref_axis',(0.,0.,-1.));
#2355=DIRECTION('',(-0.513577720619322,1.05079970984514E-16,-0.858043078687464));
#2356=DIRECTION('center_axis',(1.,0.,0.));
#2357=DIRECTION('ref_axis',(0.,0.,-1.));
#2358=DIRECTION('center_axis',(1.,0.,0.));
#2359=DIRECTION('ref_axis',(0.,0.,-1.));
#2360=DIRECTION('',(-1.,0.,0.));
#2361=DIRECTION('center_axis',(-1.,0.,0.));
#2362=DIRECTION('ref_axis',(0.,0.,-1.));
#2363=DIRECTION('',(0.983571141526098,-2.21074390598966E-17,-0.180520939386676));
#2364=DIRECTION('center_axis',(1.,0.,0.));
#2365=DIRECTION('ref_axis',(0.,0.,-1.));
#2366=DIRECTION('center_axis',(1.,0.,0.));
#2367=DIRECTION('ref_axis',(0.,0.,-1.));
#2368=DIRECTION('center_axis',(1.,0.,0.));
#2369=DIRECTION('ref_axis',(0.,0.,-1.));
#2370=DIRECTION('center_axis',(1.,0.,0.));
#2371=DIRECTION('ref_axis',(0.,0.,-1.));
#2372=DIRECTION('',(1.,0.,0.));
#4354=CARTESIAN_POINT('',(0.,0.,0.));
#4355=CARTESIAN_POINT('Origin',(-32.0305529756126,-0.749999999999998,0.));
#4356=CARTESIAN_POINT('',(-26.9411105316953,-0.749999999999998,-2.57875622086151));
#4357=CARTESIAN_POINT('',(-24.9598233877886,-0.749999999999997,-2.57875622086151));
#4358=CARTESIAN_POINT('',(-25.7922242605427,-0.749999999999997,-2.57875622086151));
#4359=CARTESIAN_POINT('',(-26.9411105316953,-0.749999999999998,-1.83684484821367));
#4360=CARTESIAN_POINT('',(-26.9411105316953,-0.749999999999998,-1.34280337788449));
#4361=CARTESIAN_POINT('',(-24.9598233877886,-0.749999999999997,-1.83684484821367));
#4362=CARTESIAN_POINT('',(-21.6665165759647,-0.749999999999997,-1.83684484821367));
#4363=CARTESIAN_POINT('',(-24.9598233877886,-0.749999999999997,0.));
#4364=CARTESIAN_POINT('Origin',(-32.0305529756126,-0.749999999999998,0.));
#4365=CARTESIAN_POINT('',(-24.9598233877886,-0.749999999999997,2.57875622086151));
#4366=CARTESIAN_POINT('',(-26.9411105316953,-0.749999999999998,2.57875622086151));
#4367=CARTESIAN_POINT('',(-25.7922242605427,-0.749999999999997,2.57875622086151));
#4368=CARTESIAN_POINT('',(-24.9598233877886,-0.749999999999997,1.83684484821367));
#4369=CARTESIAN_POINT('',(-24.9598233877886,-0.749999999999997,0.));
#4370=CARTESIAN_POINT('',(-26.9411105316953,-0.749999999999998,1.83684484821367));
#4371=CARTESIAN_POINT('',(-21.6665165759647,-0.749999999999997,1.83684484821367));
#4372=CARTESIAN_POINT('',(-26.9411105316953,-0.749999999999998,-1.34280337788449));
#4373=CARTESIAN_POINT('Origin',(-24.9598233877886,-0.0500000000000033,0.));
#4374=CARTESIAN_POINT('',(-24.6433379893901,-0.674369275830021,-2.59955952546743));
#4375=CARTESIAN_POINT('Ctrl Pts',(-24.9598233877886,-0.749999999999997,
-2.57875622086151));
#4376=CARTESIAN_POINT('Ctrl Pts',(-24.8714588989999,-0.749999999999997,
-2.57875622086151));
#4377=CARTESIAN_POINT('Ctrl Pts',(-24.7775423290656,-0.732251654012554,
-2.58411714720213));
#4378=CARTESIAN_POINT('Ctrl Pts',(-24.6751102588048,-0.689726977700767,
-2.59553646483285));
#4379=CARTESIAN_POINT('Ctrl Pts',(-24.6590554485685,-0.682336269919017,
-2.59749275377718));
#4380=CARTESIAN_POINT('Ctrl Pts',(-24.6433379893901,-0.674369275830042,
-2.59955952546742));
#4381=CARTESIAN_POINT('',(-24.2598233877886,-0.0499999999999985,-1.9834311171324));
#4382=CARTESIAN_POINT('Ctrl Pts',(-24.2598233877886,-0.0500000000000034,
-1.9834311171324));
#4383=CARTESIAN_POINT('Ctrl Pts',(-24.2598233877886,-0.139024680847254,
-1.98118690809287));
#4384=CARTESIAN_POINT('Ctrl Pts',(-24.2778228093247,-0.233283857786286,
-1.97223255425957));
#4385=CARTESIAN_POINT('Ctrl Pts',(-24.349705656948,-0.405631974937099,-1.94411555901275));
#4386=CARTESIAN_POINT('Ctrl Pts',(-24.4035428766891,-0.483787439248121,
-1.92524336790881));
#4387=CARTESIAN_POINT('Ctrl Pts',(-24.5269368573565,-0.606943918256759,
-1.89002872240561));
#4388=CARTESIAN_POINT('Ctrl Pts',(-24.6049717534738,-0.660537412507157,
-1.87126930464578));
#4389=CARTESIAN_POINT('Ctrl Pts',(-24.7769694082335,-0.732084988974823,
-1.8444538864071));
#4390=CARTESIAN_POINT('Ctrl Pts',(-24.8710178004329,-0.749999999999997,
-1.83684484821367));
#4391=CARTESIAN_POINT('Ctrl Pts',(-24.9598233877886,-0.749999999999997,
-1.83684484821367));
#4392=CARTESIAN_POINT('',(-24.2598233877886,-0.0499999999999985,-2.72441956476416));
#4393=CARTESIAN_POINT('',(-24.2598233877886,-0.0499999999999985,0.));
#4394=CARTESIAN_POINT('Ctrl Pts',(-24.6433379893901,-0.674369275830043,
-2.59955952546742));
#4395=CARTESIAN_POINT('Ctrl Pts',(-24.5848581377007,-0.64472653094067,-2.60724934991992));
#4396=CARTESIAN_POINT('Ctrl Pts',(-24.531196418248,-0.607203802215661,-2.61926288147073));
#4397=CARTESIAN_POINT('Ctrl Pts',(-24.4188018998553,-0.502917996238797,
-2.65129970036023));
#4398=CARTESIAN_POINT('Ctrl Pts',(-24.3656895097955,-0.430698662203228,
-2.67244287095924));
#4399=CARTESIAN_POINT('Ctrl Pts',(-24.2967339716088,-0.285490706378351,
-2.70312656992203));
#4400=CARTESIAN_POINT('Ctrl Pts',(-24.2758927310872,-0.215972246591974,
-2.71398152997755));
#4401=CARTESIAN_POINT('Ctrl Pts',(-24.2619469726382,-0.112808220815181,
-2.72227581593582));
#4402=CARTESIAN_POINT('Ctrl Pts',(-24.2598338408088,-0.081573716422347,
-2.72383525661314));
#4403=CARTESIAN_POINT('Ctrl Pts',(-24.2598234264347,-0.0502326037857873,
-2.72441527796272));
#4404=CARTESIAN_POINT('Ctrl Pts',(-24.2598234006703,-0.0501550682186355,
-2.72441671289213));
#4405=CARTESIAN_POINT('Ctrl Pts',(-24.2598233877886,-0.0500775336225404,
-2.7244181418258));
#4406=CARTESIAN_POINT('Ctrl Pts',(-24.2598233877886,-0.0499999999999986,
-2.72441956476417));
#4407=CARTESIAN_POINT('Origin',(-24.2598233877886,-0.0499999999999985,0.));
#4408=CARTESIAN_POINT('',(-24.2598233877886,0.0500000000000051,-2.72441956476416));
#4409=CARTESIAN_POINT('Origin',(-24.2598233877886,0.,0.));
#4410=CARTESIAN_POINT('',(-24.2598233877886,0.0500000000000051,-1.9834311171324));
#4411=CARTESIAN_POINT('Origin',(-24.2598233877886,0.,0.));
#4412=CARTESIAN_POINT('',(-24.2598233877886,0.0500000000000051,0.));
#4413=CARTESIAN_POINT('Origin',(-24.9598233877886,0.750000000000003,0.));
#4414=CARTESIAN_POINT('',(-24.9598233877886,0.750000000000003,-2.57875622086151));
#4415=CARTESIAN_POINT('',(-26.9411105316953,0.750000000000003,-2.57875622086151));
#4416=CARTESIAN_POINT('',(-25.7922242605427,0.750000000000003,-2.57875622086151));
#4417=CARTESIAN_POINT('',(-24.9598233877886,0.750000000000003,-1.83684484821366));
#4418=CARTESIAN_POINT('',(-24.9598233877886,0.750000000000003,0.));
#4419=CARTESIAN_POINT('',(-26.9411105316953,0.750000000000003,-1.83684484821366));
#4420=CARTESIAN_POINT('',(-21.6665165759647,0.750000000000004,-1.83684484821366));
#4421=CARTESIAN_POINT('',(-26.9411105316953,0.750000000000003,-1.34280337788449));
#4422=CARTESIAN_POINT('Origin',(-24.9598233877886,0.050000000000005,0.));
#4423=CARTESIAN_POINT('',(-24.6433379893901,0.674369275830023,-2.59955952546743));
#4424=CARTESIAN_POINT('Ctrl Pts',(-24.2598233877886,0.0500000000000053,
-2.72441956476417));
#4425=CARTESIAN_POINT('Ctrl Pts',(-24.2598233877886,0.0500775341306451,
-2.72441814181648));
#4426=CARTESIAN_POINT('Ctrl Pts',(-24.2598234006705,0.0501550687267315,
-2.72441671288273));
#4427=CARTESIAN_POINT('Ctrl Pts',(-24.2598234264347,0.050232603785789,-2.72441527796272));
#4428=CARTESIAN_POINT('Ctrl Pts',(-24.2598455995816,0.116960674997039,-2.72318035990581));
#4429=CARTESIAN_POINT('Ctrl Pts',(-24.2693721788655,0.182817524037613,-2.71744107277057));
#4430=CARTESIAN_POINT('Ctrl Pts',(-24.3111665384102,0.325934269006048,-2.69640279204955));
#4431=CARTESIAN_POINT('Ctrl Pts',(-24.3482258638932,0.400187099831499,-2.67924676947619));
#4432=CARTESIAN_POINT('Ctrl Pts',(-24.451725722152,0.540287158645911,-2.64091034959975));
#4433=CARTESIAN_POINT('Ctrl Pts',(-24.5211658067261,0.603472684928343,-2.61969621846221));
#4434=CARTESIAN_POINT('Ctrl Pts',(-24.615213593946,0.659505977432703,-2.60354842317404));
#4435=CARTESIAN_POINT('Ctrl Pts',(-24.6291544833972,0.667179824461095,-2.60142458955455));
#4436=CARTESIAN_POINT('Ctrl Pts',(-24.6433379893901,0.674369275830048,-2.59955952546742));
#4437=CARTESIAN_POINT('Ctrl Pts',(-24.9598233877886,0.750000000000003,-1.83684484821366));
#4438=CARTESIAN_POINT('Ctrl Pts',(-24.8710178004329,0.750000000000002,-1.83684484821366));
#4439=CARTESIAN_POINT('Ctrl Pts',(-24.7769694082335,0.732084988974827,-1.84445388640709));
#4440=CARTESIAN_POINT('Ctrl Pts',(-24.6049717534738,0.660537412507157,-1.87126930464578));
#4441=CARTESIAN_POINT('Ctrl Pts',(-24.5269368573564,0.606943918256764,-1.89002872240561));
#4442=CARTESIAN_POINT('Ctrl Pts',(-24.4035428766891,0.483787439248125,-1.92524336790881));
#4443=CARTESIAN_POINT('Ctrl Pts',(-24.349705656948,0.405631974937107,-1.94411555901275));
#4444=CARTESIAN_POINT('Ctrl Pts',(-24.2778228093247,0.233283857786291,-1.97223255425957));
#4445=CARTESIAN_POINT('Ctrl Pts',(-24.2598233877886,0.139024680847256,-1.98118690809287));
#4446=CARTESIAN_POINT('Ctrl Pts',(-24.2598233877886,0.050000000000005,-1.9834311171324));
#4447=CARTESIAN_POINT('Ctrl Pts',(-24.6433379893901,0.674369275830048,-2.59955952546742));
#4448=CARTESIAN_POINT('Ctrl Pts',(-24.6590554485685,0.682336269919023,-2.59749275377718));
#4449=CARTESIAN_POINT('Ctrl Pts',(-24.6751102588048,0.689726977700771,-2.59553646483285));
#4450=CARTESIAN_POINT('Ctrl Pts',(-24.7775423290656,0.732251654012559,-2.58411714720213));
#4451=CARTESIAN_POINT('Ctrl Pts',(-24.8714588989999,0.750000000000003,-2.57875622086151));
#4452=CARTESIAN_POINT('Ctrl Pts',(-24.9598233877886,0.750000000000003,-2.57875622086151));
#4453=CARTESIAN_POINT('Origin',(-24.9598233877886,0.750000000000003,0.));
#4454=CARTESIAN_POINT('',(-26.9411105316953,0.750000000000003,2.57875622086151));
#4455=CARTESIAN_POINT('',(-24.9598233877886,0.750000000000003,2.57875622086151));
#4456=CARTESIAN_POINT('',(-25.7922242605427,0.750000000000003,2.57875622086151));
#4457=CARTESIAN_POINT('',(-26.9411105316953,0.750000000000003,1.83684484821366));
#4458=CARTESIAN_POINT('',(-26.9411105316953,0.750000000000003,-1.34280337788449));
#4459=CARTESIAN_POINT('',(-24.9598233877886,0.750000000000003,1.83684484821366));
#4460=CARTESIAN_POINT('',(-21.6665165759647,0.750000000000004,1.83684484821366));
#4461=CARTESIAN_POINT('',(-24.9598233877886,0.750000000000003,0.));
#4462=CARTESIAN_POINT('Origin',(-24.9598233877886,0.050000000000005,0.));
#4463=CARTESIAN_POINT('',(-24.6433379893901,0.674369275830023,2.59955952546743));
#4464=CARTESIAN_POINT('',(-24.2598233877886,0.0500000000000051,2.72441956476416));
#4465=CARTESIAN_POINT('Ctrl Pts',(-24.6433379893901,0.674369275830048,2.59955952546742));
#4466=CARTESIAN_POINT('Ctrl Pts',(-24.5948713345161,0.649802101930525,2.60593266180436));
#4467=CARTESIAN_POINT('Ctrl Pts',(-24.5496532706599,0.619791430299218,2.61528239730828));
#4468=CARTESIAN_POINT('Ctrl Pts',(-24.4417200371024,0.528744950462541,2.64346770524035));
#4469=CARTESIAN_POINT('Ctrl Pts',(-24.3860923106545,0.460462041863293,2.66434536458396));
#4470=CARTESIAN_POINT('Ctrl Pts',(-24.3090437545258,0.318322152326005,2.69712526693607));
#4471=CARTESIAN_POINT('Ctrl Pts',(-24.2840037138287,0.247396071480533,2.70974202041489));
#4472=CARTESIAN_POINT('Ctrl Pts',(-24.2634679001427,0.132431551146189,2.72119842129899));
#4473=CARTESIAN_POINT('Ctrl Pts',(-24.2598233877886,0.0912752037123824,
2.72366206022548));
#4474=CARTESIAN_POINT('Ctrl Pts',(-24.2598233877886,0.0500000000000052,
2.72441956476417));
#4475=CARTESIAN_POINT('Ctrl Pts',(-24.9598233877886,0.750000000000003,2.57875622086151));
#4476=CARTESIAN_POINT('Ctrl Pts',(-24.8714588989999,0.750000000000003,2.57875622086151));
#4477=CARTESIAN_POINT('Ctrl Pts',(-24.7775423290656,0.732251654012559,2.58411714720213));
#4478=CARTESIAN_POINT('Ctrl Pts',(-24.6751102588048,0.689726977700771,2.59553646483285));
#4479=CARTESIAN_POINT('Ctrl Pts',(-24.6590554485684,0.682336269919021,2.59749275377718));
#4480=CARTESIAN_POINT('Ctrl Pts',(-24.6433379893901,0.674369275830044,2.59955952546742));
#4481=CARTESIAN_POINT('',(-24.2598233877886,0.0500000000000051,1.9834311171324));
#4482=CARTESIAN_POINT('Ctrl Pts',(-24.2598233877886,0.050000000000005,1.9834311171324));
#4483=CARTESIAN_POINT('Ctrl Pts',(-24.2598233877886,0.139024680847256,1.98118690809287));
#4484=CARTESIAN_POINT('Ctrl Pts',(-24.2778228093247,0.233283857786291,1.97223255425957));
#4485=CARTESIAN_POINT('Ctrl Pts',(-24.349705656948,0.405631974937107,1.94411555901275));
#4486=CARTESIAN_POINT('Ctrl Pts',(-24.4035428766891,0.483787439248125,1.92524336790881));
#4487=CARTESIAN_POINT('Ctrl Pts',(-24.5269368573564,0.606943918256764,1.89002872240561));
#4488=CARTESIAN_POINT('Ctrl Pts',(-24.6049717534738,0.660537412507161,1.87126930464578));
#4489=CARTESIAN_POINT('Ctrl Pts',(-24.7769694082335,0.732084988974829,1.84445388640709));
#4490=CARTESIAN_POINT('Ctrl Pts',(-24.8710178004329,0.750000000000003,1.83684484821366));
#4491=CARTESIAN_POINT('Ctrl Pts',(-24.9598233877886,0.750000000000003,1.83684484821366));
#4492=CARTESIAN_POINT('',(-24.2598233877886,0.0500000000000051,0.));
#4493=CARTESIAN_POINT('Origin',(-24.2598233877886,-0.0499999999999985,0.));
#4494=CARTESIAN_POINT('',(-24.2598233877886,-3.33701353648822E-16,2.7248783394621));
#4495=CARTESIAN_POINT('Origin',(-24.2598233877886,0.,0.));
#4496=CARTESIAN_POINT('',(-24.2598233877886,-2.4297742445139E-16,1.9840612380693));
#4497=CARTESIAN_POINT('Origin',(-24.2598233877886,0.,0.));
#4498=CARTESIAN_POINT('',(-24.2598233877886,-0.0499999999999985,1.9834311171324));
#4499=CARTESIAN_POINT('Origin',(-24.2598233877886,0.,0.));
#4500=CARTESIAN_POINT('',(-24.2598233877886,-0.0499999999999985,2.72441956476416));
#4501=CARTESIAN_POINT('',(-24.2598233877886,-0.0499999999999985,0.));
#4502=CARTESIAN_POINT('Origin',(-24.2598233877886,0.,0.));
#4503=CARTESIAN_POINT('Origin',(-24.9598233877886,-0.0500000000000033,0.));
#4504=CARTESIAN_POINT('',(-24.6433379893901,-0.674369275830021,2.59955952546743));
#4505=CARTESIAN_POINT('Ctrl Pts',(-24.6433379893901,-0.674369275830042,
2.59955952546742));
#4506=CARTESIAN_POINT('Ctrl Pts',(-24.6590554485685,-0.682336269919019,
2.59749275377718));
#4507=CARTESIAN_POINT('Ctrl Pts',(-24.6751102588048,-0.689726977700767,
2.59553646483285));
#4508=CARTESIAN_POINT('Ctrl Pts',(-24.7775423290656,-0.732251654012554,
2.58411714720213));
#4509=CARTESIAN_POINT('Ctrl Pts',(-24.8714588989999,-0.749999999999997,
2.57875622086151));
#4510=CARTESIAN_POINT('Ctrl Pts',(-24.9598233877886,-0.749999999999997,
2.57875622086151));
#4511=CARTESIAN_POINT('Ctrl Pts',(-24.2598233877886,-0.0499999999999988,
2.72441956476417));
#4512=CARTESIAN_POINT('Ctrl Pts',(-24.2598233877886,-0.104924766187127,
2.72341155617956));
#4513=CARTESIAN_POINT('Ctrl Pts',(-24.2662698540133,-0.159426953545748,
2.71936770640943));
#4514=CARTESIAN_POINT('Ctrl Pts',(-24.2974260951431,-0.28987136967753,2.7030112297106));
#4515=CARTESIAN_POINT('Ctrl Pts',(-24.3286906053069,-0.36268639361365,2.68794464981024));
#4516=CARTESIAN_POINT('Ctrl Pts',(-24.4216661799565,-0.507384818705599,
2.65103909321305));
#4517=CARTESIAN_POINT('Ctrl Pts',(-24.4879327399939,-0.575597877337425,
2.62866780596057));
#4518=CARTESIAN_POINT('Ctrl Pts',(-24.5908215755151,-0.64559465234568,2.60749770242026));
#4519=CARTESIAN_POINT('Ctrl Pts',(-24.6166208950646,-0.660826696832337,
2.60307269725752));
#4520=CARTESIAN_POINT('Ctrl Pts',(-24.6433379893901,-0.674369275830043,
2.59955952546742));
#4521=CARTESIAN_POINT('Ctrl Pts',(-24.9598233877886,-0.749999999999997,
1.83684484821367));
#4522=CARTESIAN_POINT('Ctrl Pts',(-24.8710178004329,-0.749999999999997,
1.83684484821367));
#4523=CARTESIAN_POINT('Ctrl Pts',(-24.7769694082335,-0.732084988974822,
1.8444538864071));
#4524=CARTESIAN_POINT('Ctrl Pts',(-24.6049717534738,-0.660537412507153,
1.87126930464578));
#4525=CARTESIAN_POINT('Ctrl Pts',(-24.5269368573565,-0.606943918256759,
1.89002872240561));
#4526=CARTESIAN_POINT('Ctrl Pts',(-24.4035428766891,-0.483787439248121,
1.92524336790881));
#4527=CARTESIAN_POINT('Ctrl Pts',(-24.349705656948,-0.4056319749371,1.94411555901275));
#4528=CARTESIAN_POINT('Ctrl Pts',(-24.2778228093247,-0.233283857786286,
1.97223255425957));
#4529=CARTESIAN_POINT('Ctrl Pts',(-24.2598233877886,-0.139024680847255,
1.98118690809287));
#4530=CARTESIAN_POINT('Ctrl Pts',(-24.2598233877886,-0.0500000000000034,
1.9834311171324));
#4531=CARTESIAN_POINT('Origin',(-24.6433379893901,0.,0.));
#4532=CARTESIAN_POINT('',(-23.9997961170673,-3.42705006664759E-16,2.79839874569029));
#4533=CARTESIAN_POINT('Origin',(-23.9997961170673,0.,0.));
#4534=CARTESIAN_POINT('Origin',(-24.6433379893901,-5.60629501944673E-16,
4.57788729236058));
#4535=CARTESIAN_POINT('Origin',(-24.6433379893901,0.,0.));
#4536=CARTESIAN_POINT('Origin',(-24.6433379893901,0.,0.));
#4537=CARTESIAN_POINT('Origin',(-21.6665165759647,0.,0.));
#4538=CARTESIAN_POINT('',(-16.3919226202342,-2.4297742445139E-16,1.9840612380693));
#4539=CARTESIAN_POINT('',(-21.6665165759647,-2.4297742445139E-16,1.9840612380693));
#4540=CARTESIAN_POINT('Origin',(-16.3919226202342,0.,0.));
#4541=CARTESIAN_POINT('Origin',(-26.9411105316953,0.,0.));
#4542=CARTESIAN_POINT('Origin',(-26.9411105316953,0.,0.));
#4543=CARTESIAN_POINT('Origin',(-25.7922242605427,0.,0.));
#4544=CARTESIAN_POINT('Origin',(-26.9411105316953,0.,0.));
#4545=CARTESIAN_POINT('Origin',(-25.7922242605427,0.,0.));
#4546=CARTESIAN_POINT('Origin',(-26.9411105316953,0.,0.));
#4547=CARTESIAN_POINT('Origin',(-26.9411105316953,0.,-2.68560675576897));
#4548=CARTESIAN_POINT('Origin',(-26.9411105316953,0.,-2.68560675576897));
#4549=CARTESIAN_POINT('Origin',(-16.3919226202342,0.,-1.9840612380693));
#4550=CARTESIAN_POINT('',(-16.3919226202342,-2.83677232469619E-16,2.3164003912567));
#4551=CARTESIAN_POINT('Origin',(-16.3919226202342,0.,0.));
#4552=CARTESIAN_POINT('Origin',(-23.9374740777754,0.,0.));
#4553=CARTESIAN_POINT('',(-23.8751520384835,-3.42705006664759E-16,2.79839874569029));
#4554=CARTESIAN_POINT('Origin',(-23.8751520384835,0.,0.));
#4555=CARTESIAN_POINT('',(-23.9374740777754,-3.42705006664758E-16,2.79839874569029));
#4556=CARTESIAN_POINT('Origin',(-23.8146350180683,0.,0.));
#4557=CARTESIAN_POINT('',(-23.754117997653,-3.6746903553126E-16,3.00061238707443));
#4558=CARTESIAN_POINT('Origin',(-23.754117997653,0.,0.));
#4559=CARTESIAN_POINT('',(-23.8146350180683,-3.55087021098009E-16,2.89950556638236));
#4560=CARTESIAN_POINT('Origin',(-12.0843030466866,0.,0.));
#4561=CARTESIAN_POINT('',(-0.41448809572012,-3.6746903553126E-16,3.00061238707443));
#4562=CARTESIAN_POINT('Origin',(-0.41448809572012,0.,0.));
#4563=CARTESIAN_POINT('',(-12.0843030466866,-3.6746903553126E-16,3.00061238707443));
#4564=CARTESIAN_POINT('Origin',(-0.199995922856362,0.,0.));
#4565=CARTESIAN_POINT('',(0.0144962500073953,-3.57826880652553E-16,2.92187821747206));
#4566=CARTESIAN_POINT('',(-0.199995922856362,3.62647958091906E-16,2.96124530227324));
#4567=CARTESIAN_POINT('Origin',(0.0144962500073953,0.,0.));
#4568=CARTESIAN_POINT('Origin',(0.0144962500073953,0.,-2.3164003912567));
#4569=CARTESIAN_POINT('',(0.0144962500073953,-2.83677232469619E-16,2.3164003912567));
#4570=CARTESIAN_POINT('Origin',(0.0144962500073953,0.,0.));
#4571=CARTESIAN_POINT('Origin',(-8.1887131851134,0.,0.));
#4572=CARTESIAN_POINT('',(-8.1887131851134,-2.83677232469619E-16,2.3164003912567));
#4601=UNCERTAINTY_MEASURE_WITH_UNIT(LENGTH_MEASURE(0.01),#4614,
'DISTANCE_ACCURACY_VALUE',
'Maximum model space distance between geometric entities at asserted c
onnectivities');
#4603=UNCERTAINTY_MEASURE_WITH_UNIT(LENGTH_MEASURE(0.01),#4614,
'DISTANCE_ACCURACY_VALUE',
'Maximum model space distance between geometric entities at asserted c
onnectivities');
#4611=(
GEOMETRIC_REPRESENTATION_CONTEXT(3)
GLOBAL_UNCERTAINTY_ASSIGNED_CONTEXT((#4601))
GLOBAL_UNIT_ASSIGNED_CONTEXT((#4614,#4616,#4617))
REPRESENTATION_CONTEXT('','3D')
);
#4613=(
GEOMETRIC_REPRESENTATION_CONTEXT(3)
GLOBAL_UNCERTAINTY_ASSIGNED_CONTEXT((#4603))
GLOBAL_UNIT_ASSIGNED_CONTEXT((#4614,#4616,#4617))
REPRESENTATION_CONTEXT('','3D')
);
#4614=(
LENGTH_UNIT()
NAMED_UNIT(*)
SI_UNIT(.MILLI.,.METRE.)
);
#4616=(
NAMED_UNIT(*)
PLANE_ANGLE_UNIT()
SI_UNIT($,.RADIAN.)
);
#4617=(
NAMED_UNIT(*)
SI_UNIT($,.STERADIAN.)
SOLID_ANGLE_UNIT()
);
#4625=SHAPE_DEFINITION_REPRESENTATION(#4634,#4651);
#4634=PRODUCT_DEFINITION_SHAPE('',$,#4661);
#4651=SHAPE_REPRESENTATION('',(#1841),#4611);
#4653=PRODUCT_DEFINITION_CONTEXT('part definition',#4682,'design');
#4661=PRODUCT_DEFINITION('Adjustment_Part','Adjustment_Part',#4670,#4653);
#4670=PRODUCT_DEFINITION_FORMATION('',$,#4691);
#4682=APPLICATION_CONTEXT(
'Core Data for Automotive Mechanical Design Process');
#4683=PRODUCT_CONTEXT('part definition',#4682,'mechanical');
#4691=PRODUCT('Adjustment_Part','Adjustment_Part',$,(#4683));
#4695=PRESENTATION_STYLE_ASSIGNMENT((#4700));
#4700=SURFACE_STYLE_USAGE(.BOTH.,#4705);
#4705=SURFACE_SIDE_STYLE('',(#4710));
#4710=SURFACE_STYLE_FILL_AREA(#4715);
#4715=FILL_AREA_STYLE('Opaque(255,255,255)',(#4720));
#4720=FILL_AREA_STYLE_COLOUR('Opaque(255,255,255)',#4725);
#4725=COLOUR_RGB('Opaque(255,255,255)', 0.66274510, 0.83137255, 0.94901961);
ENDSEC;
END-ISO-10303-21;
